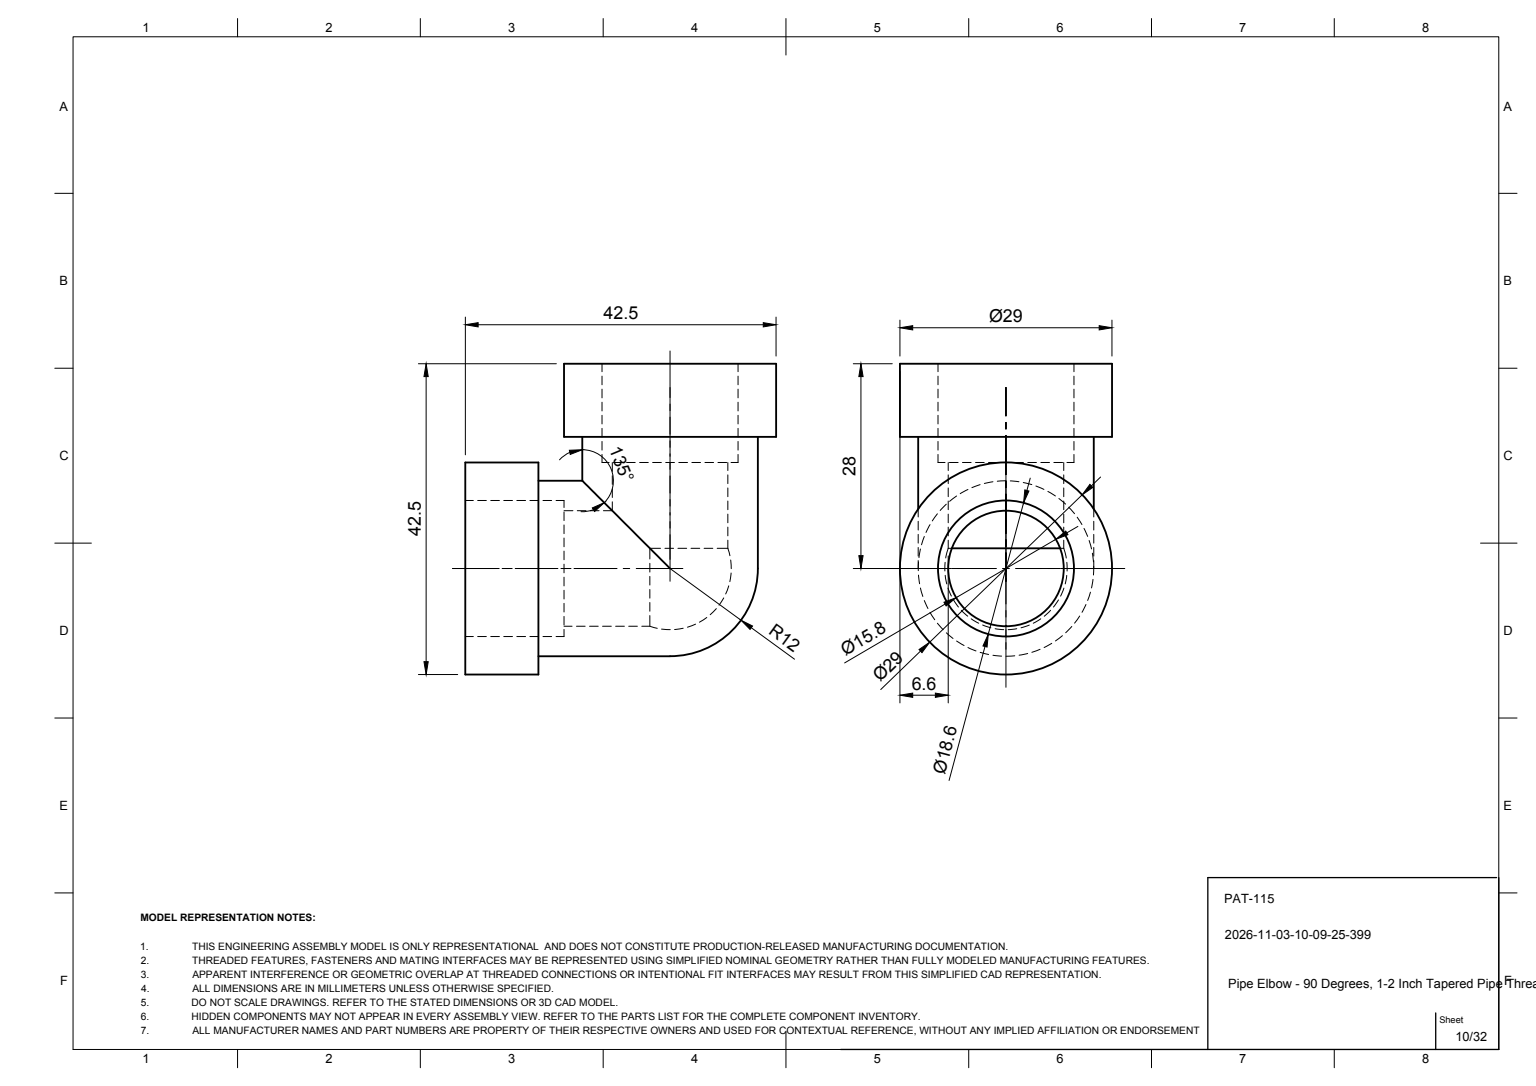
ISO-10303-21;
HEADER;
/* Generated by software containing ST-Developer
 * from STEP Tools, Inc. (www.steptools.com) 
 */

FILE_DESCRIPTION(
/* description */ ('Union bypass pipe loop'),
/* implementation_level */ '2;1');

FILE_NAME(
/* name */ 'Pipe Elbow - 90 Degrees, 1-2 Inch Tapered Pipe Thread.step',
/* time_stamp */ '2026-10-27T21:00:29-07:00',
/* author */ (''),
/* organization */ (''),
/* preprocessor_version */ 'ST-DEVELOPER v20.2',
/* originating_system */ 'Autodesk Translation Framework v15.17.0.0',
/* authorisation */ '');

FILE_SCHEMA (('AUTOMOTIVE_DESIGN { 1 0 10303 214 3 1 1 }'));
ENDSEC;

DATA;
#10=MECHANICAL_DESIGN_GEOMETRIC_PRESENTATION_REPRESENTATION('',(#464),#10095);
#25=ELLIPSE('',#6313,1.11722871427475,0.79);
#26=ELLIPSE('',#6337,1.69705627484771,1.2);
#400=SHAPE_REPRESENTATION_RELATIONSHIP('SRR','None',#10269,#432);
#432=ADVANCED_BREP_SHAPE_REPRESENTATION('',(#494),#10081);
#464=STYLED_ITEM('',(#10486),#494);
#494=MANIFOLD_SOLID_BREP('Body1',#5537);
#508=SPHERICAL_SURFACE('',#6317,0.837);
#509=SPHERICAL_SURFACE('',#6331,1.2);
#588=FACE_BOUND('',#1430,.T.);
#589=FACE_BOUND('',#1433,.T.);
#590=FACE_BOUND('',#1437,.T.);
#591=FACE_BOUND('',#1441,.T.);
#592=FACE_BOUND('',#1444,.T.);
#593=FACE_BOUND('',#1446,.T.);
#594=FACE_BOUND('',#1449,.T.);
#738=PLANE('',#6323);
#739=PLANE('',#6330);
#740=PLANE('',#6339);
#741=PLANE('',#6343);
#742=PLANE('',#6344);
#743=PLANE('',#6349);
#1019=FACE_OUTER_BOUND('',#1428,.T.);
#1020=FACE_OUTER_BOUND('',#1429,.T.);
#1021=FACE_OUTER_BOUND('',#1431,.T.);
#1022=FACE_OUTER_BOUND('',#1432,.T.);
#1023=FACE_OUTER_BOUND('',#1434,.T.);
#1024=FACE_OUTER_BOUND('',#1435,.T.);
#1025=FACE_OUTER_BOUND('',#1436,.T.);
#1026=FACE_OUTER_BOUND('',#1438,.T.);
#1027=FACE_OUTER_BOUND('',#1439,.T.);
#1028=FACE_OUTER_BOUND('',#1440,.T.);
#1029=FACE_OUTER_BOUND('',#1442,.T.);
#1030=FACE_OUTER_BOUND('',#1443,.T.);
#1031=FACE_OUTER_BOUND('',#1445,.T.);
#1032=FACE_OUTER_BOUND('',#1447,.T.);
#1033=FACE_OUTER_BOUND('',#1448,.T.);
#1034=FACE_OUTER_BOUND('',#1450,.T.);
#1428=EDGE_LOOP('',(#4476,#4477,#4478,#4479,#4480,#4481));
#1429=EDGE_LOOP('',(#4482,#4483));
#1430=EDGE_LOOP('',(#4484,#4485,#4486,#4487));
#1431=EDGE_LOOP('',(#4488,#4489,#4490,#4491,#4492,#4493));
#1432=EDGE_LOOP('',(#4494));
#1433=EDGE_LOOP('',(#4495));
#1434=EDGE_LOOP('',(#4496,#4497,#4498,#4499));
#1435=EDGE_LOOP('',(#4500,#4501,#4502,#4503));
#1436=EDGE_LOOP('',(#4504));
#1437=EDGE_LOOP('',(#4505));
#1438=EDGE_LOOP('',(#4506,#4507,#4508,#4509));
#1439=EDGE_LOOP('',(#4510,#4511,#4512,#4513,#4514,#4515));
#1440=EDGE_LOOP('',(#4516));
#1441=EDGE_LOOP('',(#4517));
#1442=EDGE_LOOP('',(#4518,#4519,#4520,#4521));
#1443=EDGE_LOOP('',(#4522));
#1444=EDGE_LOOP('',(#4523));
#1445=EDGE_LOOP('',(#4524));
#1446=EDGE_LOOP('',(#4525));
#1447=EDGE_LOOP('',(#4526,#4527,#4528,#4529));
#1448=EDGE_LOOP('',(#4530));
#1449=EDGE_LOOP('',(#4531));
#1450=EDGE_LOOP('',(#4532,#4533,#4534,#4535,#4536,#4537));
#1815=LINE('',#9305,#2191);
#1816=LINE('',#9317,#2192);
#1817=LINE('',#9325,#2193);
#1818=LINE('',#9330,#2194);
#1819=LINE('',#9345,#2195);
#1820=LINE('',#9353,#2196);
#1821=LINE('',#9363,#2197);
#1822=LINE('',#9366,#2198);
#2191=VECTOR('',#7631,0.79);
#2192=VECTOR('',#7646,0.79);
#2193=VECTOR('',#7657,0.93);
#2194=VECTOR('',#7662,0.93);
#2195=VECTOR('',#7681,1.2);
#2196=VECTOR('',#7692,1.45);
#2197=VECTOR('',#7705,1.45);
#2198=VECTOR('',#7710,1.2);
#2526=CIRCLE('',#6314,0.79);
#2527=CIRCLE('',#6315,0.79);
#2528=CIRCLE('',#6316,0.79);
#2529=CIRCLE('',#6318,0.837);
#2530=CIRCLE('',#6319,0.79);
#2531=CIRCLE('',#6320,0.79);
#2532=CIRCLE('',#6322,0.79);
#2533=CIRCLE('',#6324,0.93);
#2534=CIRCLE('',#6326,0.93);
#2535=CIRCLE('',#6328,0.93);
#2536=CIRCLE('',#6329,0.93);
#2537=CIRCLE('',#6332,1.2);
#2538=CIRCLE('',#6333,1.2);
#2539=CIRCLE('',#6334,1.2);
#2540=CIRCLE('',#6335,1.2);
#2541=CIRCLE('',#6338,1.2);
#2542=CIRCLE('',#6340,1.45);
#2543=CIRCLE('',#6342,1.45);
#2544=CIRCLE('',#6345,1.45);
#2545=CIRCLE('',#6346,1.2);
#2546=CIRCLE('',#6348,1.45);
#2870=VERTEX_POINT('',#9299);
#2871=VERTEX_POINT('',#9300);
#2872=VERTEX_POINT('',#9302);
#2873=VERTEX_POINT('',#9304);
#2874=VERTEX_POINT('',#9309);
#2875=VERTEX_POINT('',#9310);
#2876=VERTEX_POINT('',#9312);
#2877=VERTEX_POINT('',#9316);
#2878=VERTEX_POINT('',#9320);
#2879=VERTEX_POINT('',#9323);
#2880=VERTEX_POINT('',#9327);
#2881=VERTEX_POINT('',#9329);
#2882=VERTEX_POINT('',#9334);
#2883=VERTEX_POINT('',#9335);
#2884=VERTEX_POINT('',#9337);
#2885=VERTEX_POINT('',#9339);
#2886=VERTEX_POINT('',#9344);
#2887=VERTEX_POINT('',#9348);
#2888=VERTEX_POINT('',#9351);
#2889=VERTEX_POINT('',#9356);
#2890=VERTEX_POINT('',#9358);
#2891=VERTEX_POINT('',#9361);
#3436=EDGE_CURVE('',#2870,#2871,#25,.T.);
#3437=EDGE_CURVE('',#2872,#2870,#2526,.T.);
#3438=EDGE_CURVE('',#2872,#2873,#1815,.T.);
#3439=EDGE_CURVE('',#2873,#2873,#2527,.T.);
#3440=EDGE_CURVE('',#2871,#2872,#2528,.T.);
#3441=EDGE_CURVE('',#2874,#2875,#2529,.T.);
#3442=EDGE_CURVE('',#2870,#2876,#2530,.T.);
#3443=EDGE_CURVE('',#2876,#2871,#2531,.T.);
#3444=EDGE_CURVE('',#2876,#2877,#1816,.T.);
#3445=EDGE_CURVE('',#2877,#2877,#2532,.T.);
#3446=EDGE_CURVE('',#2878,#2878,#2533,.T.);
#3447=EDGE_CURVE('',#2879,#2879,#2534,.T.);
#3448=EDGE_CURVE('',#2879,#2878,#1817,.T.);
#3449=EDGE_CURVE('',#2880,#2880,#2535,.T.);
#3450=EDGE_CURVE('',#2880,#2881,#1818,.T.);
#3451=EDGE_CURVE('',#2881,#2881,#2536,.T.);
#3452=EDGE_CURVE('',#2882,#2883,#2537,.T.);
#3453=EDGE_CURVE('',#2883,#2884,#2538,.T.);
#3454=EDGE_CURVE('',#2885,#2884,#2539,.T.);
#3455=EDGE_CURVE('',#2882,#2885,#2540,.T.);
#3456=EDGE_CURVE('',#2884,#2882,#26,.T.);
#3457=EDGE_CURVE('',#2883,#2886,#1819,.T.);
#3458=EDGE_CURVE('',#2886,#2886,#2541,.T.);
#3459=EDGE_CURVE('',#2887,#2887,#2542,.T.);
#3460=EDGE_CURVE('',#2888,#2888,#2543,.T.);
#3461=EDGE_CURVE('',#2888,#2887,#1820,.T.);
#3462=EDGE_CURVE('',#2889,#2889,#2544,.T.);
#3463=EDGE_CURVE('',#2890,#2890,#2545,.T.);
#3464=EDGE_CURVE('',#2891,#2891,#2546,.T.);
#3465=EDGE_CURVE('',#2891,#2889,#1821,.T.);
#3466=EDGE_CURVE('',#2890,#2885,#1822,.T.);
#4476=ORIENTED_EDGE('',*,*,#3436,.F.);
#4477=ORIENTED_EDGE('',*,*,#3437,.F.);
#4478=ORIENTED_EDGE('',*,*,#3438,.T.);
#4479=ORIENTED_EDGE('',*,*,#3439,.F.);
#4480=ORIENTED_EDGE('',*,*,#3438,.F.);
#4481=ORIENTED_EDGE('',*,*,#3440,.F.);
#4482=ORIENTED_EDGE('',*,*,#3441,.T.);
#4483=ORIENTED_EDGE('',*,*,#3441,.F.);
#4484=ORIENTED_EDGE('',*,*,#3440,.T.);
#4485=ORIENTED_EDGE('',*,*,#3437,.T.);
#4486=ORIENTED_EDGE('',*,*,#3442,.T.);
#4487=ORIENTED_EDGE('',*,*,#3443,.T.);
#4488=ORIENTED_EDGE('',*,*,#3436,.T.);
#4489=ORIENTED_EDGE('',*,*,#3443,.F.);
#4490=ORIENTED_EDGE('',*,*,#3444,.T.);
#4491=ORIENTED_EDGE('',*,*,#3445,.F.);
#4492=ORIENTED_EDGE('',*,*,#3444,.F.);
#4493=ORIENTED_EDGE('',*,*,#3442,.F.);
#4494=ORIENTED_EDGE('',*,*,#3446,.F.);
#4495=ORIENTED_EDGE('',*,*,#3439,.T.);
#4496=ORIENTED_EDGE('',*,*,#3447,.F.);
#4497=ORIENTED_EDGE('',*,*,#3448,.T.);
#4498=ORIENTED_EDGE('',*,*,#3446,.T.);
#4499=ORIENTED_EDGE('',*,*,#3448,.F.);
#4500=ORIENTED_EDGE('',*,*,#3449,.F.);
#4501=ORIENTED_EDGE('',*,*,#3450,.T.);
#4502=ORIENTED_EDGE('',*,*,#3451,.F.);
#4503=ORIENTED_EDGE('',*,*,#3450,.F.);
#4504=ORIENTED_EDGE('',*,*,#3449,.T.);
#4505=ORIENTED_EDGE('',*,*,#3445,.T.);
#4506=ORIENTED_EDGE('',*,*,#3452,.T.);
#4507=ORIENTED_EDGE('',*,*,#3453,.T.);
#4508=ORIENTED_EDGE('',*,*,#3454,.F.);
#4509=ORIENTED_EDGE('',*,*,#3455,.F.);
#4510=ORIENTED_EDGE('',*,*,#3456,.F.);
#4511=ORIENTED_EDGE('',*,*,#3453,.F.);
#4512=ORIENTED_EDGE('',*,*,#3457,.T.);
#4513=ORIENTED_EDGE('',*,*,#3458,.T.);
#4514=ORIENTED_EDGE('',*,*,#3457,.F.);
#4515=ORIENTED_EDGE('',*,*,#3452,.F.);
#4516=ORIENTED_EDGE('',*,*,#3459,.F.);
#4517=ORIENTED_EDGE('',*,*,#3447,.T.);
#4518=ORIENTED_EDGE('',*,*,#3460,.F.);
#4519=ORIENTED_EDGE('',*,*,#3461,.T.);
#4520=ORIENTED_EDGE('',*,*,#3459,.T.);
#4521=ORIENTED_EDGE('',*,*,#3461,.F.);
#4522=ORIENTED_EDGE('',*,*,#3460,.T.);
#4523=ORIENTED_EDGE('',*,*,#3458,.F.);
#4524=ORIENTED_EDGE('',*,*,#3462,.F.);
#4525=ORIENTED_EDGE('',*,*,#3463,.T.);
#4526=ORIENTED_EDGE('',*,*,#3464,.F.);
#4527=ORIENTED_EDGE('',*,*,#3465,.T.);
#4528=ORIENTED_EDGE('',*,*,#3462,.T.);
#4529=ORIENTED_EDGE('',*,*,#3465,.F.);
#4530=ORIENTED_EDGE('',*,*,#3464,.T.);
#4531=ORIENTED_EDGE('',*,*,#3451,.T.);
#4532=ORIENTED_EDGE('',*,*,#3463,.F.);
#4533=ORIENTED_EDGE('',*,*,#3466,.T.);
#4534=ORIENTED_EDGE('',*,*,#3454,.T.);
#4535=ORIENTED_EDGE('',*,*,#3456,.T.);
#4536=ORIENTED_EDGE('',*,*,#3455,.T.);
#4537=ORIENTED_EDGE('',*,*,#3466,.F.);
#5147=CYLINDRICAL_SURFACE('',#6312,0.79);
#5148=CYLINDRICAL_SURFACE('',#6321,0.79);
#5149=CYLINDRICAL_SURFACE('',#6325,0.93);
#5150=CYLINDRICAL_SURFACE('',#6327,0.93);
#5151=CYLINDRICAL_SURFACE('',#6336,1.2);
#5152=CYLINDRICAL_SURFACE('',#6341,1.45);
#5153=CYLINDRICAL_SURFACE('',#6347,1.45);
#5154=CYLINDRICAL_SURFACE('',#6350,1.2);
#5368=ADVANCED_FACE('',(#1019),#5147,.F.);
#5369=ADVANCED_FACE('',(#1020,#588),#508,.F.);
#5370=ADVANCED_FACE('',(#1021),#5148,.F.);
#5371=ADVANCED_FACE('',(#1022,#589),#738,.F.);
#5372=ADVANCED_FACE('',(#1023),#5149,.F.);
#5373=ADVANCED_FACE('',(#1024),#5150,.F.);
#5374=ADVANCED_FACE('',(#1025,#590),#739,.F.);
#5375=ADVANCED_FACE('',(#1026),#509,.T.);
#5376=ADVANCED_FACE('',(#1027),#5151,.T.);
#5377=ADVANCED_FACE('',(#1028,#591),#740,.T.);
#5378=ADVANCED_FACE('',(#1029),#5152,.T.);
#5379=ADVANCED_FACE('',(#1030,#592),#741,.T.);
#5380=ADVANCED_FACE('',(#1031,#593),#742,.T.);
#5381=ADVANCED_FACE('',(#1032),#5153,.T.);
#5382=ADVANCED_FACE('',(#1033,#594),#743,.T.);
#5383=ADVANCED_FACE('',(#1034),#5154,.T.);
#5537=CLOSED_SHELL('',(#5368,#5369,#5370,#5371,#5372,#5373,#5374,#5375,
#5376,#5377,#5378,#5379,#5380,#5381,#5382,#5383));
#6311=AXIS2_PLACEMENT_3D('',#9297,#7623,#7624);
#6312=AXIS2_PLACEMENT_3D('',#9298,#7625,#7626);
#6313=AXIS2_PLACEMENT_3D('',#9301,#7627,#7628);
#6314=AXIS2_PLACEMENT_3D('',#9303,#7629,#7630);
#6315=AXIS2_PLACEMENT_3D('',#9306,#7632,#7633);
#6316=AXIS2_PLACEMENT_3D('',#9307,#7634,#7635);
#6317=AXIS2_PLACEMENT_3D('',#9308,#7636,#7637);
#6318=AXIS2_PLACEMENT_3D('',#9311,#7638,#7639);
#6319=AXIS2_PLACEMENT_3D('',#9313,#7640,#7641);
#6320=AXIS2_PLACEMENT_3D('',#9314,#7642,#7643);
#6321=AXIS2_PLACEMENT_3D('',#9315,#7644,#7645);
#6322=AXIS2_PLACEMENT_3D('',#9318,#7647,#7648);
#6323=AXIS2_PLACEMENT_3D('',#9319,#7649,#7650);
#6324=AXIS2_PLACEMENT_3D('',#9321,#7651,#7652);
#6325=AXIS2_PLACEMENT_3D('',#9322,#7653,#7654);
#6326=AXIS2_PLACEMENT_3D('',#9324,#7655,#7656);
#6327=AXIS2_PLACEMENT_3D('',#9326,#7658,#7659);
#6328=AXIS2_PLACEMENT_3D('',#9328,#7660,#7661);
#6329=AXIS2_PLACEMENT_3D('',#9331,#7663,#7664);
#6330=AXIS2_PLACEMENT_3D('',#9332,#7665,#7666);
#6331=AXIS2_PLACEMENT_3D('',#9333,#7667,#7668);
#6332=AXIS2_PLACEMENT_3D('',#9336,#7669,#7670);
#6333=AXIS2_PLACEMENT_3D('',#9338,#7671,#7672);
#6334=AXIS2_PLACEMENT_3D('',#9340,#7673,#7674);
#6335=AXIS2_PLACEMENT_3D('',#9341,#7675,#7676);
#6336=AXIS2_PLACEMENT_3D('',#9342,#7677,#7678);
#6337=AXIS2_PLACEMENT_3D('',#9343,#7679,#7680);
#6338=AXIS2_PLACEMENT_3D('',#9346,#7682,#7683);
#6339=AXIS2_PLACEMENT_3D('',#9347,#7684,#7685);
#6340=AXIS2_PLACEMENT_3D('',#9349,#7686,#7687);
#6341=AXIS2_PLACEMENT_3D('',#9350,#7688,#7689);
#6342=AXIS2_PLACEMENT_3D('',#9352,#7690,#7691);
#6343=AXIS2_PLACEMENT_3D('',#9354,#7693,#7694);
#6344=AXIS2_PLACEMENT_3D('',#9355,#7695,#7696);
#6345=AXIS2_PLACEMENT_3D('',#9357,#7697,#7698);
#6346=AXIS2_PLACEMENT_3D('',#9359,#7699,#7700);
#6347=AXIS2_PLACEMENT_3D('',#9360,#7701,#7702);
#6348=AXIS2_PLACEMENT_3D('',#9362,#7703,#7704);
#6349=AXIS2_PLACEMENT_3D('',#9364,#7706,#7707);
#6350=AXIS2_PLACEMENT_3D('',#9365,#7708,#7709);
#7623=DIRECTION('axis',(0.,0.,1.));
#7624=DIRECTION('refdir',(1.,0.,0.));
#7625=DIRECTION('center_axis',(0.,1.,0.));
#7626=DIRECTION('ref_axis',(1.,0.,0.));
#7627=DIRECTION('center_axis',(-0.707106781186548,0.707106781186548,0.));
#7628=DIRECTION('ref_axis',(0.707106781186547,0.707106781186547,0.));
#7629=DIRECTION('center_axis',(0.,1.,0.));
#7630=DIRECTION('ref_axis',(1.,0.,0.));
#7631=DIRECTION('',(0.,1.,0.));
#7632=DIRECTION('center_axis',(0.,-1.,0.));
#7633=DIRECTION('ref_axis',(1.,0.,0.));
#7634=DIRECTION('center_axis',(0.,1.,0.));
#7635=DIRECTION('ref_axis',(1.,0.,0.));
#7636=DIRECTION('center_axis',(6.12323399573677E-17,0.,1.));
#7637=DIRECTION('ref_axis',(1.,0.,0.));
#7638=DIRECTION('center_axis',(-1.22464679914735E-16,1.,0.));
#7639=DIRECTION('ref_axis',(-1.,-1.22464679914735E-16,0.));
#7640=DIRECTION('center_axis',(1.,0.,0.));
#7641=DIRECTION('ref_axis',(0.,0.,-1.));
#7642=DIRECTION('center_axis',(1.,0.,0.));
#7643=DIRECTION('ref_axis',(0.,0.,-1.));
#7644=DIRECTION('center_axis',(1.,0.,0.));
#7645=DIRECTION('ref_axis',(0.,0.,-1.));
#7646=DIRECTION('',(1.,0.,0.));
#7647=DIRECTION('center_axis',(-1.,0.,0.));
#7648=DIRECTION('ref_axis',(0.,0.,-1.));
#7649=DIRECTION('center_axis',(0.,-1.,0.));
#7650=DIRECTION('ref_axis',(0.,0.,-1.));
#7651=DIRECTION('center_axis',(0.,-1.,0.));
#7652=DIRECTION('ref_axis',(1.,0.,0.));
#7653=DIRECTION('center_axis',(0.,-1.,0.));
#7654=DIRECTION('ref_axis',(1.,0.,0.));
#7655=DIRECTION('center_axis',(0.,-1.,0.));
#7656=DIRECTION('ref_axis',(1.,0.,0.));
#7657=DIRECTION('',(0.,-1.,0.));
#7658=DIRECTION('center_axis',(1.,0.,0.));
#7659=DIRECTION('ref_axis',(0.,1.,0.));
#7660=DIRECTION('center_axis',(1.,0.,0.));
#7661=DIRECTION('ref_axis',(0.,0.,-1.));
#7662=DIRECTION('',(1.,0.,0.));
#7663=DIRECTION('center_axis',(-1.,0.,0.));
#7664=DIRECTION('ref_axis',(0.,1.,0.));
#7665=DIRECTION('center_axis',(-1.,0.,0.));
#7666=DIRECTION('ref_axis',(0.,0.,1.));
#7667=DIRECTION('center_axis',(6.12323399573677E-17,0.,1.));
#7668=DIRECTION('ref_axis',(1.,0.,0.));
#7669=DIRECTION('center_axis',(0.,-1.,0.));
#7670=DIRECTION('ref_axis',(1.,0.,0.));
#7671=DIRECTION('center_axis',(0.,-1.,0.));
#7672=DIRECTION('ref_axis',(1.,0.,0.));
#7673=DIRECTION('center_axis',(1.,0.,0.));
#7674=DIRECTION('ref_axis',(0.,0.,-1.));
#7675=DIRECTION('center_axis',(1.,0.,0.));
#7676=DIRECTION('ref_axis',(0.,0.,-1.));
#7677=DIRECTION('center_axis',(0.,-1.,0.));
#7678=DIRECTION('ref_axis',(1.,0.,0.));
#7679=DIRECTION('center_axis',(0.707106781186548,-0.707106781186548,0.));
#7680=DIRECTION('ref_axis',(0.707106781186547,0.707106781186547,0.));
#7681=DIRECTION('',(0.,1.,0.));
#7682=DIRECTION('center_axis',(0.,-1.,0.));
#7683=DIRECTION('ref_axis',(1.,0.,0.));
#7684=DIRECTION('center_axis',(0.,1.,0.));
#7685=DIRECTION('ref_axis',(0.,0.,1.));
#7686=DIRECTION('center_axis',(0.,-1.,0.));
#7687=DIRECTION('ref_axis',(1.,0.,0.));
#7688=DIRECTION('center_axis',(0.,-1.,0.));
#7689=DIRECTION('ref_axis',(1.,0.,0.));
#7690=DIRECTION('center_axis',(0.,-1.,0.));
#7691=DIRECTION('ref_axis',(1.,0.,0.));
#7692=DIRECTION('',(0.,1.,0.));
#7693=DIRECTION('center_axis',(0.,-1.,0.));
#7694=DIRECTION('ref_axis',(0.,0.,-1.));
#7695=DIRECTION('center_axis',(-1.,0.,0.));
#7696=DIRECTION('ref_axis',(0.,0.,1.));
#7697=DIRECTION('center_axis',(1.,0.,0.));
#7698=DIRECTION('ref_axis',(0.,0.,-1.));
#7699=DIRECTION('center_axis',(1.,0.,0.));
#7700=DIRECTION('ref_axis',(0.,0.,-1.));
#7701=DIRECTION('center_axis',(1.,0.,0.));
#7702=DIRECTION('ref_axis',(0.,1.,0.));
#7703=DIRECTION('center_axis',(1.,0.,0.));
#7704=DIRECTION('ref_axis',(0.,0.,-1.));
#7705=DIRECTION('',(-1.,0.,0.));
#7706=DIRECTION('center_axis',(1.,0.,0.));
#7707=DIRECTION('ref_axis',(0.,0.,-1.));
#7708=DIRECTION('center_axis',(1.,0.,0.));
#7709=DIRECTION('ref_axis',(0.,1.,0.));
#7710=DIRECTION('',(-1.,0.,0.));
#9297=CARTESIAN_POINT('',(0.,0.,0.));
#9298=CARTESIAN_POINT('Origin',(0.,0.,0.));
#9299=CARTESIAN_POINT('',(0.276530287672074,0.276530287672074,0.740020945649513));
#9300=CARTESIAN_POINT('',(0.276530287672074,0.276530287672074,-0.740020945649513));
#9301=CARTESIAN_POINT('Origin',(0.,0.,0.));
#9302=CARTESIAN_POINT('',(-0.79,0.276530287672074,9.67470971326409E-17));
#9303=CARTESIAN_POINT('Origin',(0.,0.276530287672074,0.));
#9304=CARTESIAN_POINT('',(-0.79,1.45,-9.67470971326409E-17));
#9305=CARTESIAN_POINT('',(-0.79,0.,9.67470971326409E-17));
#9306=CARTESIAN_POINT('Origin',(0.,1.45,0.));
#9307=CARTESIAN_POINT('Origin',(0.,0.276530287672074,0.));
#9308=CARTESIAN_POINT('Origin',(0.,0.,0.));
#9309=CARTESIAN_POINT('',(-5.12514685443167E-17,-6.27649469043988E-33,-0.837));
#9310=CARTESIAN_POINT('',(-5.12514685443167E-17,-6.27649469043988E-33,0.837));
#9311=CARTESIAN_POINT('Origin',(0.,0.,0.));
#9312=CARTESIAN_POINT('',(0.276530287672074,-9.67470971326409E-17,0.79));
#9313=CARTESIAN_POINT('Origin',(0.276530287672074,0.,0.));
#9314=CARTESIAN_POINT('Origin',(0.276530287672074,0.,0.));
#9315=CARTESIAN_POINT('Origin',(0.,0.,0.));
#9316=CARTESIAN_POINT('',(1.45,9.67470971326409E-17,0.79));
#9317=CARTESIAN_POINT('',(0.,-9.67470971326409E-17,0.79));
#9318=CARTESIAN_POINT('Origin',(1.45,0.,0.));
#9319=CARTESIAN_POINT('Origin',(0.,1.45,0.));
#9320=CARTESIAN_POINT('',(-0.93,1.45,-1.13892152320704E-16));
#9321=CARTESIAN_POINT('Origin',(0.,1.45,0.));
#9322=CARTESIAN_POINT('Origin',(0.,2.175,0.));
#9323=CARTESIAN_POINT('',(-0.93,2.8,-1.13892152320704E-16));
#9324=CARTESIAN_POINT('Origin',(0.,2.8,0.));
#9325=CARTESIAN_POINT('',(-0.93,2.175,-1.13892152320704E-16));
#9326=CARTESIAN_POINT('Origin',(2.175,0.,0.));
#9327=CARTESIAN_POINT('',(1.45,-0.93,-1.13892152320704E-16));
#9328=CARTESIAN_POINT('Origin',(1.45,0.,0.));
#9329=CARTESIAN_POINT('',(2.8,-0.93,1.13892152320704E-16));
#9330=CARTESIAN_POINT('',(2.175,-0.93,-1.13892152320704E-16));
#9331=CARTESIAN_POINT('Origin',(2.8,0.,0.));
#9332=CARTESIAN_POINT('Origin',(1.45,0.93,0.));
#9333=CARTESIAN_POINT('Origin',(0.,0.,0.));
#9334=CARTESIAN_POINT('',(0.,0.,1.2));
#9335=CARTESIAN_POINT('',(-1.2,1.11022302462516E-16,-1.46957615897682E-16));
#9336=CARTESIAN_POINT('Origin',(0.,0.,0.));
#9337=CARTESIAN_POINT('',(0.,0.,-1.2));
#9338=CARTESIAN_POINT('Origin',(0.,0.,0.));
#9339=CARTESIAN_POINT('',(1.11022302462516E-16,-1.2,-1.46957615897682E-16));
#9340=CARTESIAN_POINT('Origin',(0.,0.,0.));
#9341=CARTESIAN_POINT('Origin',(0.,0.,0.));
#9342=CARTESIAN_POINT('Origin',(0.,0.9,0.));
#9343=CARTESIAN_POINT('Origin',(0.,0.,0.));
#9344=CARTESIAN_POINT('',(-1.2,1.8,-1.46957615897682E-16));
#9345=CARTESIAN_POINT('',(-1.2,0.9,-1.46957615897682E-16));
#9346=CARTESIAN_POINT('Origin',(0.,1.8,0.));
#9347=CARTESIAN_POINT('Origin',(1.45,2.8,0.));
#9348=CARTESIAN_POINT('',(-1.45,2.8,-1.77573785876366E-16));
#9349=CARTESIAN_POINT('Origin',(0.,2.8,0.));
#9350=CARTESIAN_POINT('Origin',(0.,2.3,0.));
#9351=CARTESIAN_POINT('',(-1.45,1.8,-1.77573785876366E-16));
#9352=CARTESIAN_POINT('Origin',(0.,1.8,0.));
#9353=CARTESIAN_POINT('',(-1.45,2.3,-1.77573785876366E-16));
#9354=CARTESIAN_POINT('Origin',(1.2,1.8,0.));
#9355=CARTESIAN_POINT('Origin',(1.8,1.45,0.));
#9356=CARTESIAN_POINT('',(1.8,-1.45,-1.77573785876366E-16));
#9357=CARTESIAN_POINT('Origin',(1.8,0.,0.));
#9358=CARTESIAN_POINT('',(1.8,-1.2,-1.46957615897682E-16));
#9359=CARTESIAN_POINT('Origin',(1.8,0.,0.));
#9360=CARTESIAN_POINT('Origin',(2.3,0.,0.));
#9361=CARTESIAN_POINT('',(2.8,-1.45,-1.77573785876366E-16));
#9362=CARTESIAN_POINT('Origin',(2.8,0.,0.));
#9363=CARTESIAN_POINT('',(2.3,-1.45,-1.77573785876366E-16));
#9364=CARTESIAN_POINT('Origin',(2.8,0.,0.));
#9365=CARTESIAN_POINT('Origin',(0.9,0.,0.));
#9366=CARTESIAN_POINT('',(0.9,-1.2,-1.46957615897682E-16));
#10044=UNCERTAINTY_MEASURE_WITH_UNIT(LENGTH_MEASURE(0.001),#10096,
'DISTANCE_ACCURACY_VALUE',
'Maximum model space distance between geometric entities at asserted c
onnectivities');
#10058=UNCERTAINTY_MEASURE_WITH_UNIT(LENGTH_MEASURE(0.001),#10096,
'DISTANCE_ACCURACY_VALUE',
'Maximum model space distance between geometric entities at asserted c
onnectivities');
#10081=(
GEOMETRIC_REPRESENTATION_CONTEXT(3)
GLOBAL_UNCERTAINTY_ASSIGNED_CONTEXT((#10044))
GLOBAL_UNIT_ASSIGNED_CONTEXT((#10096,#10098,#10099))
REPRESENTATION_CONTEXT('','3D')
);
#10095=(
GEOMETRIC_REPRESENTATION_CONTEXT(3)
GLOBAL_UNCERTAINTY_ASSIGNED_CONTEXT((#10058))
GLOBAL_UNIT_ASSIGNED_CONTEXT((#10096,#10098,#10099))
REPRESENTATION_CONTEXT('','3D')
);
#10096=(
LENGTH_UNIT()
NAMED_UNIT(*)
SI_UNIT(.CENTI.,.METRE.)
);
#10098=(
NAMED_UNIT(*)
PLANE_ANGLE_UNIT()
SI_UNIT($,.RADIAN.)
);
#10099=(
NAMED_UNIT(*)
SI_UNIT($,.STERADIAN.)
SOLID_ANGLE_UNIT()
);
#10122=SHAPE_DEFINITION_REPRESENTATION(#10193,#10269);
#10193=PRODUCT_DEFINITION_SHAPE('',$,#10306);
#10269=SHAPE_REPRESENTATION('',(#6311),#10081);
#10283=PRODUCT_DEFINITION_CONTEXT('part definition',#10393,'design');
#10306=PRODUCT_DEFINITION(
'Pipe Elbow - 90 Degrees, 1-2 Inch Tapered Pipe Thread',
'Pipe Elbow - 90 Degrees, 1-2 Inch Tapered Pipe Thread',#10342,#10283);
#10342=PRODUCT_DEFINITION_FORMATION('',$,#10417);
#10393=APPLICATION_CONTEXT(
'Core Data for Automotive Mechanical Design Process');
#10394=PRODUCT_CONTEXT('part definition',#10393,'mechanical');
#10417=PRODUCT('Pipe Elbow - 90 Degrees, 1-2 Inch Tapered Pipe Thread',
'Pipe Elbow - 90 Degrees, 1-2 Inch Tapered Pipe Thread',
'Pipe Elbow - 90 Degrees, 1-2 Inch Tapered Pipe Thread',(#10394));
#10480=COLOUR_RGB('Light Blue',0.38,0.62,0.78);
#10481=FILL_AREA_STYLE_COLOUR('',#10480);
#10482=FILL_AREA_STYLE('',(#10481));
#10483=SURFACE_STYLE_FILL_AREA(#10482);
#10484=SURFACE_SIDE_STYLE('',(#10483));
#10485=SURFACE_STYLE_USAGE(.BOTH.,#10484);
#10486=PRESENTATION_STYLE_ASSIGNMENT((#10485));
ENDSEC;
END-ISO-10303-21;
